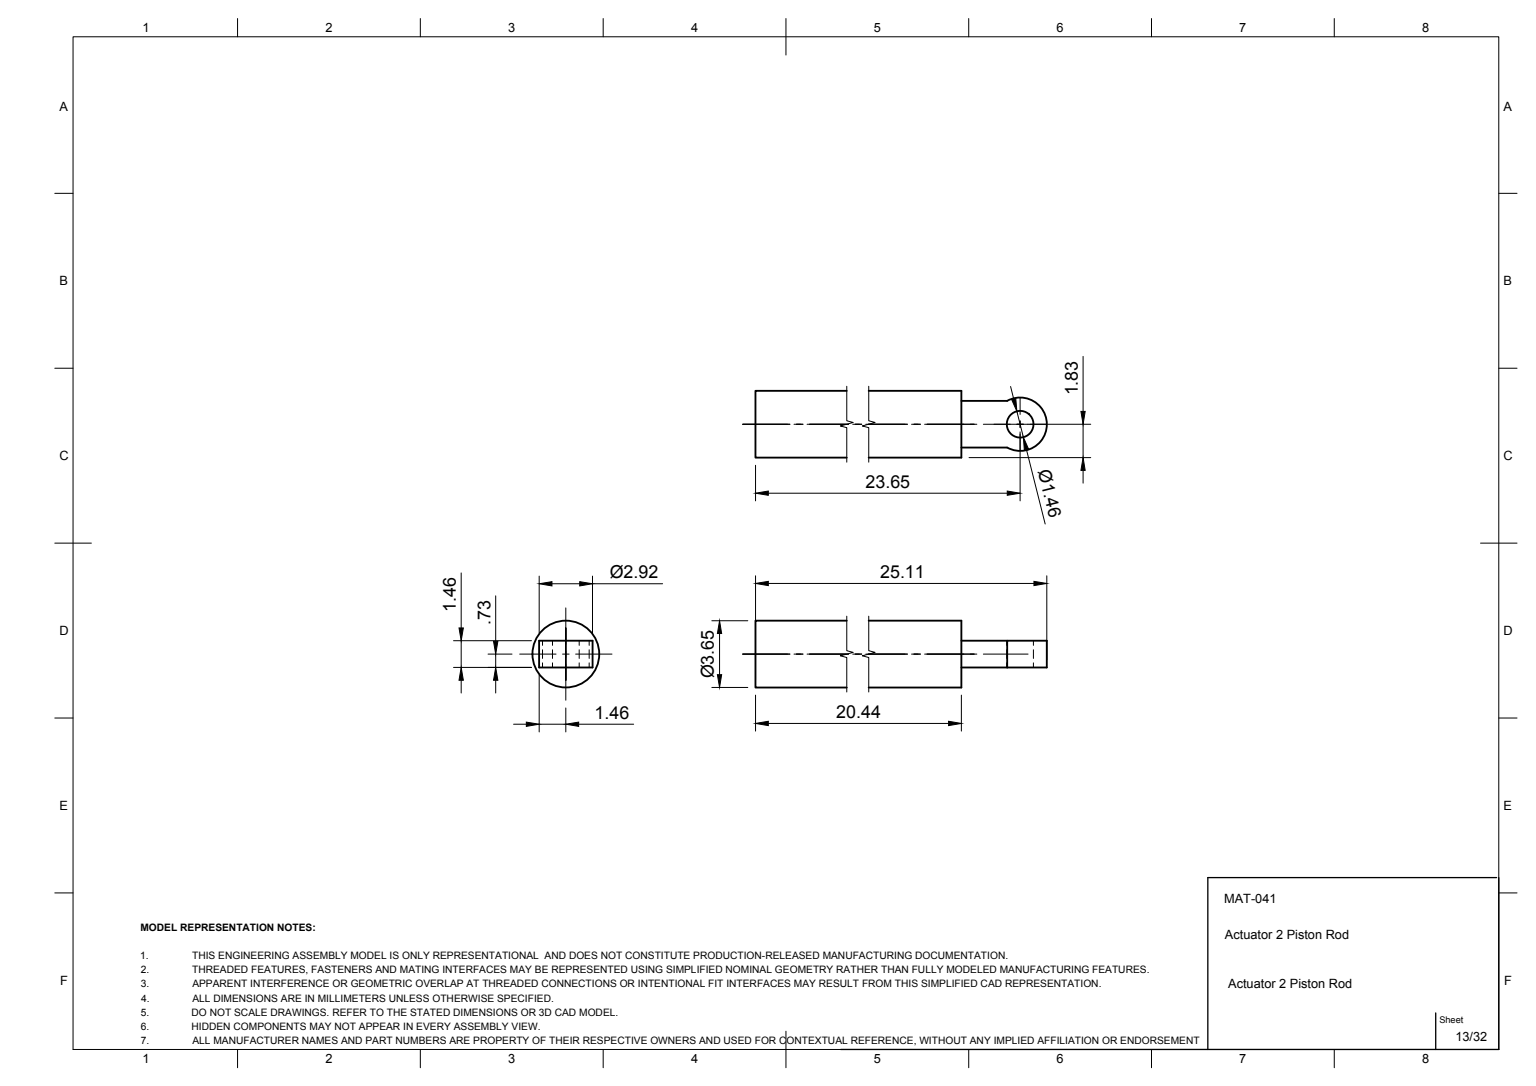
ISO-10303-21;
HEADER;
/* Generated by software containing ST-Developer
 * from STEP Tools, Inc. (www.steptools.com) 
 */

FILE_DESCRIPTION(
/* description */ ('STEP AP214'),
/* implementation_level */ '2;1');

FILE_NAME(
/* name */ 'Actuator 2 Piston Rod.step',
/* time_stamp */ '2026-11-14T21:57:47-08:00',
/* author */ (''),
/* organization */ (''),
/* preprocessor_version */ 'ST-DEVELOPER v20.2',
/* originating_system */ 'Autodesk Translation Framework v15.17.0.0',
/* authorisation */ '');

FILE_SCHEMA (('AUTOMOTIVE_DESIGN { 1 0 10303 214 3 1 1 }'));
ENDSEC;

DATA;
#10=MECHANICAL_DESIGN_GEOMETRIC_PRESENTATION_REPRESENTATION('',(#253),#13199);
#217=SHAPE_REPRESENTATION_RELATIONSHIP('SRR','None',#13286,#235);
#235=ADVANCED_BREP_SHAPE_REPRESENTATION('',(#271),#13182);
#253=STYLED_ITEM('',(#13409),#271);
#271=MANIFOLD_SOLID_BREP('Body1',#6848);
#328=FACE_BOUND('',#2448,.T.);
#329=FACE_BOUND('',#2451,.T.);
#330=FACE_BOUND('',#2454,.T.);
#492=PLANE('',#7484);
#493=PLANE('',#7485);
#494=PLANE('',#7486);
#495=PLANE('',#7487);
#496=PLANE('',#7488);
#497=PLANE('',#7489);
#873=LINE('',#11639,#1391);
#874=LINE('',#11646,#1392);
#875=LINE('',#11649,#1393);
#876=LINE('',#11654,#1394);
#877=LINE('',#11659,#1395);
#878=LINE('',#11661,#1396);
#879=LINE('',#11663,#1397);
#880=LINE('',#11664,#1398);
#881=LINE('',#11667,#1399);
#882=LINE('',#11668,#1400);
#883=LINE('',#11670,#1401);
#884=LINE('',#11672,#1402);
#1391=VECTOR('',#8926,0.729999999999999);
#1392=VECTOR('',#8933,1000.);
#1393=VECTOR('',#8936,1000.);
#1394=VECTOR('',#8941,1.825);
#1395=VECTOR('',#8946,1000.);
#1396=VECTOR('',#8947,1000.);
#1397=VECTOR('',#8948,1000.);
#1398=VECTOR('',#8949,1000.);
#1399=VECTOR('',#8954,1000.);
#1400=VECTOR('',#8955,1000.);
#1401=VECTOR('',#8958,1000.);
#1402=VECTOR('',#8961,1000.);
#1734=CYLINDRICAL_SURFACE('',#7475,0.729999999999999);
#1735=CYLINDRICAL_SURFACE('',#7478,1.46);
#1736=CYLINDRICAL_SURFACE('',#7481,1.825);
#2009=FACE_OUTER_BOUND('',#2444,.T.);
#2010=FACE_OUTER_BOUND('',#2445,.T.);
#2011=FACE_OUTER_BOUND('',#2446,.T.);
#2012=FACE_OUTER_BOUND('',#2447,.T.);
#2013=FACE_OUTER_BOUND('',#2449,.T.);
#2014=FACE_OUTER_BOUND('',#2450,.T.);
#2015=FACE_OUTER_BOUND('',#2452,.T.);
#2016=FACE_OUTER_BOUND('',#2453,.T.);
#2017=FACE_OUTER_BOUND('',#2455,.T.);
#2444=EDGE_LOOP('',(#5592,#5593,#5594,#5595));
#2445=EDGE_LOOP('',(#5596,#5597,#5598,#5599));
#2446=EDGE_LOOP('',(#5600,#5601,#5602,#5603));
#2447=EDGE_LOOP('',(#5604));
#2448=EDGE_LOOP('',(#5605,#5606,#5607,#5608));
#2449=EDGE_LOOP('',(#5609));
#2450=EDGE_LOOP('',(#5610,#5611,#5612,#5613));
#2451=EDGE_LOOP('',(#5614));
#2452=EDGE_LOOP('',(#5615,#5616,#5617,#5618));
#2453=EDGE_LOOP('',(#5619,#5620,#5621,#5622));
#2454=EDGE_LOOP('',(#5623));
#2455=EDGE_LOOP('',(#5624,#5625,#5626,#5627));
#2869=CIRCLE('',#7476,0.729999999999999);
#2870=CIRCLE('',#7477,0.729999999999999);
#2871=CIRCLE('',#7479,1.46);
#2872=CIRCLE('',#7480,1.46);
#2873=CIRCLE('',#7482,1.825);
#2874=CIRCLE('',#7483,1.825);
#3332=VERTEX_POINT('',#11636);
#3333=VERTEX_POINT('',#11638);
#3334=VERTEX_POINT('',#11642);
#3335=VERTEX_POINT('',#11643);
#3336=VERTEX_POINT('',#11645);
#3337=VERTEX_POINT('',#11647);
#3338=VERTEX_POINT('',#11651);
#3339=VERTEX_POINT('',#11653);
#3340=VERTEX_POINT('',#11657);
#3341=VERTEX_POINT('',#11658);
#3342=VERTEX_POINT('',#11660);
#3343=VERTEX_POINT('',#11662);
#4133=EDGE_CURVE('',#3332,#3332,#2869,.T.);
#4134=EDGE_CURVE('',#3332,#3333,#873,.T.);
#4135=EDGE_CURVE('',#3333,#3333,#2870,.T.);
#4136=EDGE_CURVE('',#3334,#3335,#2871,.T.);
#4137=EDGE_CURVE('',#3336,#3334,#874,.T.);
#4138=EDGE_CURVE('',#3337,#3336,#2872,.T.);
#4139=EDGE_CURVE('',#3335,#3337,#875,.T.);
#4140=EDGE_CURVE('',#3338,#3338,#2873,.T.);
#4141=EDGE_CURVE('',#3338,#3339,#876,.T.);
#4142=EDGE_CURVE('',#3339,#3339,#2874,.T.);
#4143=EDGE_CURVE('',#3340,#3341,#877,.T.);
#4144=EDGE_CURVE('',#3342,#3340,#878,.T.);
#4145=EDGE_CURVE('',#3343,#3342,#879,.T.);
#4146=EDGE_CURVE('',#3341,#3343,#880,.T.);
#4147=EDGE_CURVE('',#3337,#3340,#881,.T.);
#4148=EDGE_CURVE('',#3336,#3342,#882,.T.);
#4149=EDGE_CURVE('',#3335,#3341,#883,.T.);
#4150=EDGE_CURVE('',#3334,#3343,#884,.T.);
#5592=ORIENTED_EDGE('',*,*,#4133,.F.);
#5593=ORIENTED_EDGE('',*,*,#4134,.T.);
#5594=ORIENTED_EDGE('',*,*,#4135,.T.);
#5595=ORIENTED_EDGE('',*,*,#4134,.F.);
#5596=ORIENTED_EDGE('',*,*,#4136,.F.);
#5597=ORIENTED_EDGE('',*,*,#4137,.F.);
#5598=ORIENTED_EDGE('',*,*,#4138,.F.);
#5599=ORIENTED_EDGE('',*,*,#4139,.F.);
#5600=ORIENTED_EDGE('',*,*,#4140,.T.);
#5601=ORIENTED_EDGE('',*,*,#4141,.T.);
#5602=ORIENTED_EDGE('',*,*,#4142,.F.);
#5603=ORIENTED_EDGE('',*,*,#4141,.F.);
#5604=ORIENTED_EDGE('',*,*,#4142,.T.);
#5605=ORIENTED_EDGE('',*,*,#4143,.F.);
#5606=ORIENTED_EDGE('',*,*,#4144,.F.);
#5607=ORIENTED_EDGE('',*,*,#4145,.F.);
#5608=ORIENTED_EDGE('',*,*,#4146,.F.);
#5609=ORIENTED_EDGE('',*,*,#4140,.F.);
#5610=ORIENTED_EDGE('',*,*,#4147,.F.);
#5611=ORIENTED_EDGE('',*,*,#4138,.T.);
#5612=ORIENTED_EDGE('',*,*,#4148,.T.);
#5613=ORIENTED_EDGE('',*,*,#4144,.T.);
#5614=ORIENTED_EDGE('',*,*,#4135,.F.);
#5615=ORIENTED_EDGE('',*,*,#4149,.F.);
#5616=ORIENTED_EDGE('',*,*,#4139,.T.);
#5617=ORIENTED_EDGE('',*,*,#4147,.T.);
#5618=ORIENTED_EDGE('',*,*,#4143,.T.);
#5619=ORIENTED_EDGE('',*,*,#4136,.T.);
#5620=ORIENTED_EDGE('',*,*,#4149,.T.);
#5621=ORIENTED_EDGE('',*,*,#4146,.T.);
#5622=ORIENTED_EDGE('',*,*,#4150,.F.);
#5623=ORIENTED_EDGE('',*,*,#4133,.T.);
#5624=ORIENTED_EDGE('',*,*,#4148,.F.);
#5625=ORIENTED_EDGE('',*,*,#4137,.T.);
#5626=ORIENTED_EDGE('',*,*,#4150,.T.);
#5627=ORIENTED_EDGE('',*,*,#4145,.T.);
#6661=ADVANCED_FACE('',(#2009),#1734,.F.);
#6662=ADVANCED_FACE('',(#2010),#1735,.T.);
#6663=ADVANCED_FACE('',(#2011),#1736,.T.);
#6664=ADVANCED_FACE('',(#2012,#328),#492,.T.);
#6665=ADVANCED_FACE('',(#2013),#493,.F.);
#6666=ADVANCED_FACE('',(#2014,#329),#494,.F.);
#6667=ADVANCED_FACE('',(#2015),#495,.F.);
#6668=ADVANCED_FACE('',(#2016,#330),#496,.F.);
#6669=ADVANCED_FACE('',(#2017),#497,.F.);
#6848=CLOSED_SHELL('',(#6661,#6662,#6663,#6664,#6665,#6666,#6667,#6668,
#6669));
#7474=AXIS2_PLACEMENT_3D('',#11634,#8920,#8921);
#7475=AXIS2_PLACEMENT_3D('',#11635,#8922,#8923);
#7476=AXIS2_PLACEMENT_3D('',#11637,#8924,#8925);
#7477=AXIS2_PLACEMENT_3D('',#11640,#8927,#8928);
#7478=AXIS2_PLACEMENT_3D('',#11641,#8929,#8930);
#7479=AXIS2_PLACEMENT_3D('',#11644,#8931,#8932);
#7480=AXIS2_PLACEMENT_3D('',#11648,#8934,#8935);
#7481=AXIS2_PLACEMENT_3D('',#11650,#8937,#8938);
#7482=AXIS2_PLACEMENT_3D('',#11652,#8939,#8940);
#7483=AXIS2_PLACEMENT_3D('',#11655,#8942,#8943);
#7484=AXIS2_PLACEMENT_3D('',#11656,#8944,#8945);
#7485=AXIS2_PLACEMENT_3D('',#11665,#8950,#8951);
#7486=AXIS2_PLACEMENT_3D('',#11666,#8952,#8953);
#7487=AXIS2_PLACEMENT_3D('',#11669,#8956,#8957);
#7488=AXIS2_PLACEMENT_3D('',#11671,#8959,#8960);
#7489=AXIS2_PLACEMENT_3D('',#11673,#8962,#8963);
#8920=DIRECTION('axis',(0.,0.,1.));
#8921=DIRECTION('refdir',(1.,0.,0.));
#8922=DIRECTION('center_axis',(1.,1.23908819712629E-16,0.));
#8923=DIRECTION('ref_axis',(-1.23908819712629E-16,1.,0.));
#8924=DIRECTION('center_axis',(1.,1.23908819712629E-16,0.));
#8925=DIRECTION('ref_axis',(-1.23908819712629E-16,1.,0.));
#8926=DIRECTION('',(1.,1.23908819712629E-16,0.));
#8927=DIRECTION('center_axis',(1.,1.23908819712629E-16,0.));
#8928=DIRECTION('ref_axis',(-1.23908819712629E-16,1.,0.));
#8929=DIRECTION('center_axis',(1.,1.23908819712629E-16,0.));
#8930=DIRECTION('ref_axis',(-2.11060815823259E-32,6.12323399573677E-17,
1.));
#8931=DIRECTION('center_axis',(-1.,-1.23908819712629E-16,0.));
#8932=DIRECTION('ref_axis',(-1.23908819712629E-16,1.,0.));
#8933=DIRECTION('',(-1.,-1.23908819712629E-16,0.));
#8934=DIRECTION('center_axis',(1.,1.23908819712629E-16,0.));
#8935=DIRECTION('ref_axis',(-1.23908819712629E-16,1.,0.));
#8936=DIRECTION('',(1.,1.23908819712629E-16,0.));
#8937=DIRECTION('center_axis',(0.,0.,-1.));
#8938=DIRECTION('ref_axis',(-1.,0.,0.));
#8939=DIRECTION('center_axis',(0.,0.,1.));
#8940=DIRECTION('ref_axis',(1.,0.,0.));
#8941=DIRECTION('',(0.,0.,1.));
#8942=DIRECTION('center_axis',(0.,0.,1.));
#8943=DIRECTION('ref_axis',(1.,0.,0.));
#8944=DIRECTION('center_axis',(0.,0.,1.));
#8945=DIRECTION('ref_axis',(1.,0.,0.));
#8946=DIRECTION('',(-1.,0.,0.));
#8947=DIRECTION('',(-1.23908819712629E-16,1.,0.));
#8948=DIRECTION('',(1.,0.,0.));
#8949=DIRECTION('',(1.23908819712629E-16,-1.,0.));
#8950=DIRECTION('center_axis',(0.,0.,1.));
#8951=DIRECTION('ref_axis',(1.,0.,0.));
#8952=DIRECTION('center_axis',(-1.,-1.23908819712629E-16,0.));
#8953=DIRECTION('ref_axis',(1.23908819712629E-16,-1.,0.));
#8954=DIRECTION('',(0.,0.,-1.));
#8955=DIRECTION('',(0.,0.,-1.));
#8956=DIRECTION('center_axis',(0.,-1.,0.));
#8957=DIRECTION('ref_axis',(0.,0.,-1.));
#8958=DIRECTION('',(0.,0.,-1.));
#8959=DIRECTION('center_axis',(1.,1.23908819712629E-16,0.));
#8960=DIRECTION('ref_axis',(-1.23908819712629E-16,1.,0.));
#8961=DIRECTION('',(0.,0.,-1.));
#8962=DIRECTION('center_axis',(0.,1.,0.));
#8963=DIRECTION('ref_axis',(0.,0.,1.));
#11634=CARTESIAN_POINT('',(0.,0.,0.));
#11635=CARTESIAN_POINT('Origin',(-0.73,-4.33680868994202E-16,23.652));
#11636=CARTESIAN_POINT('',(-0.73,-0.729999999999999,23.652));
#11637=CARTESIAN_POINT('Origin',(-0.73,-4.33680868994202E-16,23.652));
#11638=CARTESIAN_POINT('',(0.73,-0.729999999999999,23.652));
#11639=CARTESIAN_POINT('',(-0.73,-0.729999999999999,23.652));
#11640=CARTESIAN_POINT('Origin',(0.73,0.,23.652));
#11641=CARTESIAN_POINT('Origin',(-4.85950360212944,-8.67361737988404E-16,
23.652));
#11642=CARTESIAN_POINT('',(-0.73,-1.2775,22.9451805393171));
#11643=CARTESIAN_POINT('',(-0.73,1.2775,22.9451805393171));
#11644=CARTESIAN_POINT('Origin',(-0.73,-4.33680868994202E-16,23.652));
#11645=CARTESIAN_POINT('',(0.73,-1.2775,22.9451805393171));
#11646=CARTESIAN_POINT('',(-4.85950360212944,-1.2775,22.9451805393171));
#11647=CARTESIAN_POINT('',(0.73,1.2775,22.9451805393171));
#11648=CARTESIAN_POINT('Origin',(0.73,0.,23.652));
#11649=CARTESIAN_POINT('',(-4.85950360212944,1.2775,22.9451805393172));
#11650=CARTESIAN_POINT('Origin',(0.,0.,20.44));
#11651=CARTESIAN_POINT('',(1.825,-2.23498040844392E-16,0.));
#11652=CARTESIAN_POINT('Origin',(0.,0.,0.));
#11653=CARTESIAN_POINT('',(1.825,-2.23498040844392E-16,20.44));
#11654=CARTESIAN_POINT('',(1.825,-2.23498040844392E-16,20.44));
#11655=CARTESIAN_POINT('Origin',(0.,0.,20.44));
#11656=CARTESIAN_POINT('Origin',(0.,0.,20.44));
#11657=CARTESIAN_POINT('',(0.73,1.2775,20.44));
#11658=CARTESIAN_POINT('',(-0.73,1.2775,20.44));
#11659=CARTESIAN_POINT('',(-0.73,1.2775,20.44));
#11660=CARTESIAN_POINT('',(0.73,-1.2775,20.44));
#11661=CARTESIAN_POINT('',(0.73,1.2775,20.44));
#11662=CARTESIAN_POINT('',(-0.73,-1.2775,20.44));
#11663=CARTESIAN_POINT('',(-0.73,-1.2775,20.44));
#11664=CARTESIAN_POINT('',(-0.73,1.2775,20.44));
#11665=CARTESIAN_POINT('Origin',(0.,0.,0.));
#11666=CARTESIAN_POINT('Origin',(0.73,1.2775,23.652));
#11667=CARTESIAN_POINT('',(0.73,1.2775,23.652));
#11668=CARTESIAN_POINT('',(0.73,-1.2775,23.652));
#11669=CARTESIAN_POINT('Origin',(-0.73,1.2775,23.652));
#11670=CARTESIAN_POINT('',(-0.73,1.2775,23.652));
#11671=CARTESIAN_POINT('Origin',(-0.73,1.2775,23.652));
#11672=CARTESIAN_POINT('',(-0.73,-1.2775,23.652));
#11673=CARTESIAN_POINT('Origin',(-0.73,-1.2775,23.652));
#13156=UNCERTAINTY_MEASURE_WITH_UNIT(LENGTH_MEASURE(0.01),#13200,
'DISTANCE_ACCURACY_VALUE',
'Maximum model space distance between geometric entities at asserted c
onnectivities');
#13173=UNCERTAINTY_MEASURE_WITH_UNIT(LENGTH_MEASURE(0.01),#13200,
'DISTANCE_ACCURACY_VALUE',
'Maximum model space distance between geometric entities at asserted c
onnectivities');
#13182=(
GEOMETRIC_REPRESENTATION_CONTEXT(3)
GLOBAL_UNCERTAINTY_ASSIGNED_CONTEXT((#13156))
GLOBAL_UNIT_ASSIGNED_CONTEXT((#13200,#13202,#13203))
REPRESENTATION_CONTEXT('','3D')
);
#13199=(
GEOMETRIC_REPRESENTATION_CONTEXT(3)
GLOBAL_UNCERTAINTY_ASSIGNED_CONTEXT((#13173))
GLOBAL_UNIT_ASSIGNED_CONTEXT((#13200,#13202,#13203))
REPRESENTATION_CONTEXT('','3D')
);
#13200=(
LENGTH_UNIT()
NAMED_UNIT(*)
SI_UNIT(.MILLI.,.METRE.)
);
#13202=(
NAMED_UNIT(*)
PLANE_ANGLE_UNIT()
SI_UNIT($,.RADIAN.)
);
#13203=(
NAMED_UNIT(*)
SI_UNIT($,.STERADIAN.)
SOLID_ANGLE_UNIT()
);
#13212=SHAPE_DEFINITION_REPRESENTATION(#13237,#13286);
#13237=PRODUCT_DEFINITION_SHAPE('',$,#13312);
#13286=SHAPE_REPRESENTATION('',(#7474),#13182);
#13303=PRODUCT_DEFINITION_CONTEXT('part definition',#13380,'design');
#13312=PRODUCT_DEFINITION('Actuator 2 Piston Rod',
'Actuator 2 Piston Rod',#13337,#13303);
#13337=PRODUCT_DEFINITION_FORMATION('',$,#13390);
#13380=APPLICATION_CONTEXT(
'Core Data for Automotive Mechanical Design Process');
#13381=PRODUCT_CONTEXT('part definition',#13380,'mechanical');
#13390=PRODUCT('Actuator 2 Piston Rod','Actuator 2 Piston Rod',$,(#13381));
#13409=PRESENTATION_STYLE_ASSIGNMENT((#13414));
#13414=SURFACE_STYLE_USAGE(.BOTH.,#13419);
#13419=SURFACE_SIDE_STYLE('',(#13424));
#13424=SURFACE_STYLE_FILL_AREA(#13429);
#13429=FILL_AREA_STYLE('Opaque(61,176,222)',(#13434));
#13434=FILL_AREA_STYLE_COLOUR('Opaque(61,176,222)',#13439);
#13439=COLOUR_RGB('Opaque(61,176,222)',0.23921568627451,0.690196078431373,
0.870588235294118);
ENDSEC;
END-ISO-10303-21;
